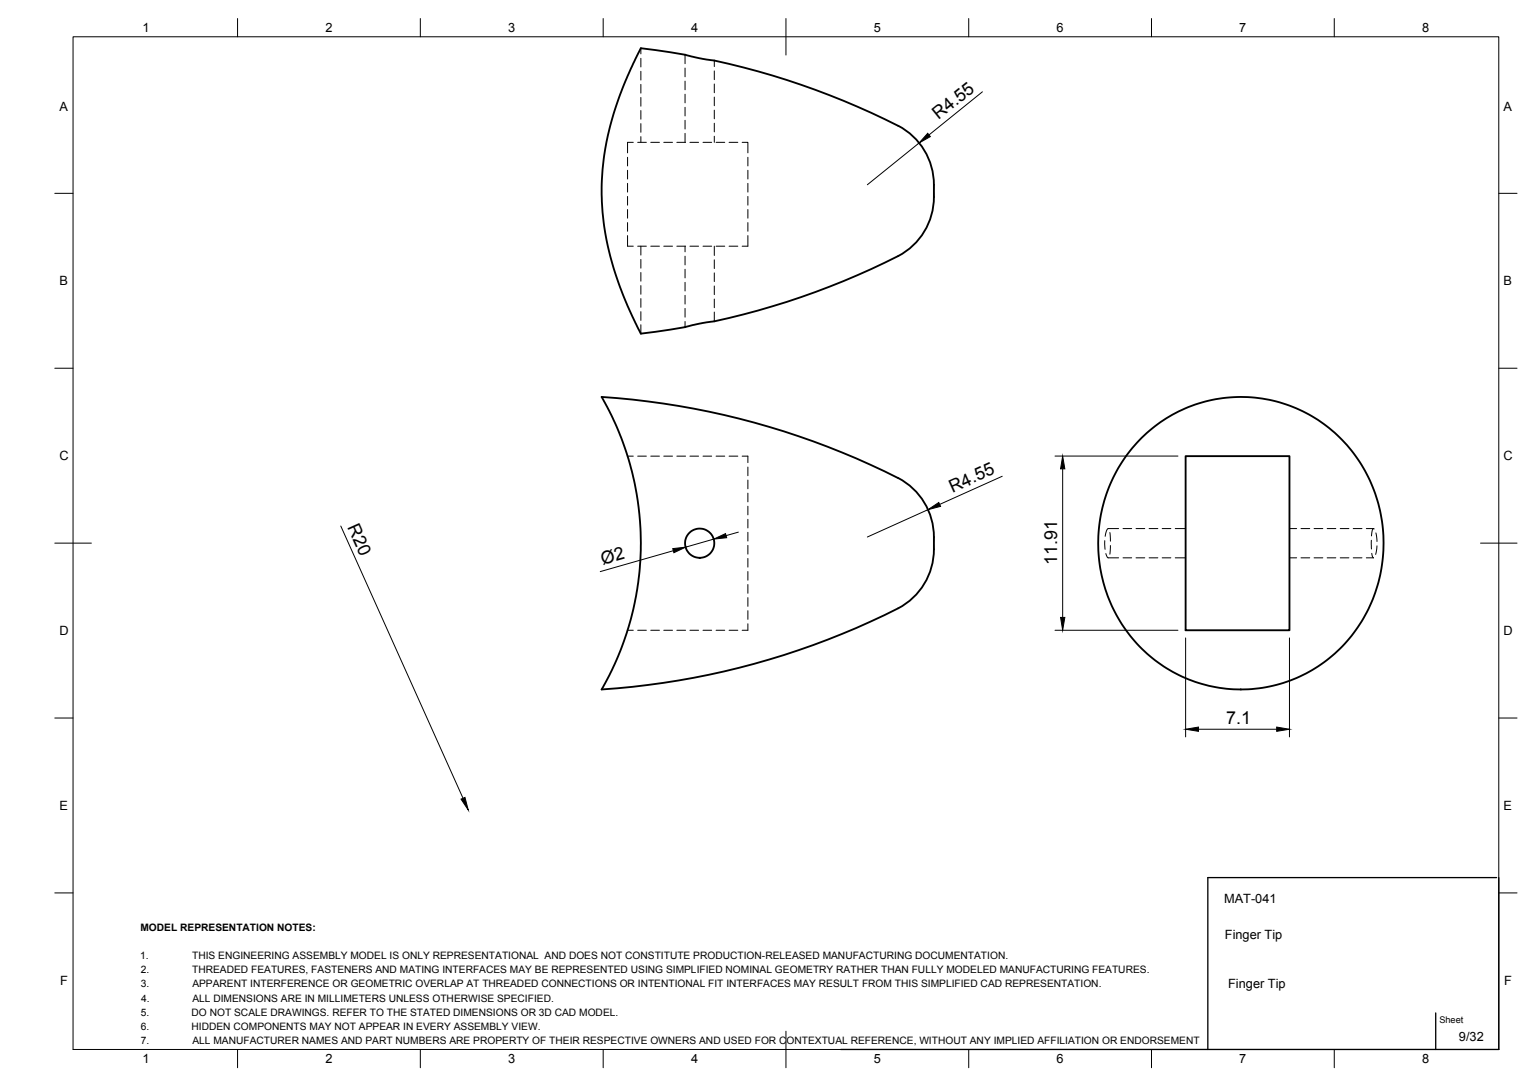
ISO-10303-21;
HEADER;
/* Generated by software containing ST-Developer
 * from STEP Tools, Inc. (www.steptools.com) 
 */

FILE_DESCRIPTION(
/* description */ ('STEP AP214'),
/* implementation_level */ '2;1');

FILE_NAME(
/* name */ 'Finger Tip.step',
/* time_stamp */ '2026-11-14T21:57:47-08:00',
/* author */ (''),
/* organization */ (''),
/* preprocessor_version */ 'ST-DEVELOPER v20.2',
/* originating_system */ 'Autodesk Translation Framework v15.17.0.0',
/* authorisation */ '');

FILE_SCHEMA (('AUTOMOTIVE_DESIGN { 1 0 10303 214 3 1 1 }'));
ENDSEC;

DATA;
#10=MECHANICAL_DESIGN_GEOMETRIC_PRESENTATION_REPRESENTATION('',(#259),#13199);
#11=(
BOUNDED_CURVE()
B_SPLINE_CURVE(2,(#12139,#12140,#12141),.UNSPECIFIED.,.F.,.F.)
B_SPLINE_CURVE_WITH_KNOTS((3,3),(0.0658194535624849,0.468554524158603),
 .UNSPECIFIED.)
CURVE()
GEOMETRIC_REPRESENTATION_ITEM()
RATIONAL_B_SPLINE_CURVE((0.999935484054137,0.979761934520674,1.))
REPRESENTATION_ITEM('')
);
#17=(
BOUNDED_SURFACE()
B_SPLINE_SURFACE(2,2,((#12039,#12040,#12041,#12042,#12043,#12044,#12045,
#12046,#12047),(#12048,#12049,#12050,#12051,#12052,#12053,#12054,#12055,
#12056),(#12057,#12058,#12059,#12060,#12061,#12062,#12063,#12064,#12065)),
 .UNSPECIFIED.,.F.,.T.,.F.)
B_SPLINE_SURFACE_WITH_KNOTS((3,3),(3,2,2,2,3),(-1.66348996389916,-0.482485072527983),
(-3.14159265358979,-1.5707963267949,0.,1.5707963267949,3.14159265358979),
 .UNSPECIFIED.)
GEOMETRIC_REPRESENTATION_ITEM()
RATIONAL_B_SPLINE_SURFACE(((1.,0.707106781186548,1.,0.707106781186548,1.,
0.707106781186548,1.,0.707106781186548,1.),(0.830661033030149,0.587366049323041,
0.830661033030149,0.587366049323041,0.830661033030149,0.587366049323041,
0.830661033030149,0.587366049323041,0.830661033030149),(1.,0.707106781186548,
1.,0.707106781186548,1.,0.707106781186548,1.,0.707106781186548,1.)))
REPRESENTATION_ITEM('')
SURFACE()
);
#18=(
BOUNDED_SURFACE()
B_SPLINE_SURFACE(2,2,((#12070,#12071,#12072,#12073,#12074,#12075,#12076,
#12077,#12078),(#12079,#12080,#12081,#12082,#12083,#12084,#12085,#12086,
#12087),(#12088,#12089,#12090,#12091,#12092,#12093,#12094,#12095,#12096)),
 .UNSPECIFIED.,.F.,.T.,.F.)
B_SPLINE_SURFACE_WITH_KNOTS((3,3),(3,2,2,2,3),(-0.468554524158603,-0.0651764989564067),
(-3.14159265358979,-1.5707963267949,0.,1.5707963267949,3.14159265358979),
 .UNSPECIFIED.)
GEOMETRIC_REPRESENTATION_ITEM()
RATIONAL_B_SPLINE_SURFACE(((1.,0.707106781186548,1.,0.707106781186548,1.,
0.707106781186548,1.,0.707106781186548,1.),(0.979729625048845,0.692773461601392,
0.979729625048845,0.692773461601392,0.979729625048845,0.692773461601392,
0.979729625048845,0.692773461601392,0.979729625048845),(1.,0.707106781186548,
1.,0.707106781186548,1.,0.707106781186548,1.,0.707106781186548,1.)))
REPRESENTATION_ITEM('')
SURFACE()
);
#184=B_SPLINE_CURVE_WITH_KNOTS('',3,(#11947,#11948,#11949,#11950,#11951,
#11952,#11953,#11954,#11955,#11956,#11957,#11958,#11959,#11960,#11961,#11962,
#11963,#11964,#11965,#11966,#11967,#11968,#11969),.UNSPECIFIED.,.F.,.F.,
(4,2,2,2,2,3,2,2,2,2,4),(0.476645491037206,0.489023957516382,0.527166589495669,
0.568095012367448,0.607142264956957,0.636252225893218,0.674200453389387,
0.713373161852222,0.750226922703377,0.78797801482852,0.795881712617993),
 .UNSPECIFIED.);
#185=B_SPLINE_CURVE_WITH_KNOTS('',3,(#11970,#11971,#11972,#11973,#11974,
#11975,#11976,#11977,#11978,#11979,#11980,#11981,#11982,#11983,#11984,#11985,
#11986,#11987,#11988,#11989),.UNSPECIFIED.,.F.,.F.,(4,2,2,2,2,2,2,2,2,4),
(0.159629486724776,0.18739470215505,0.223766252646954,0.263805807870951,
0.302029537123351,0.34097527431584,0.380812071035441,0.417115871073174,
0.453232846571769,0.476645491037206),.UNSPECIFIED.);
#186=B_SPLINE_CURVE_WITH_KNOTS('',3,(#11993,#11994,#11995,#11996,#11997,
#11998,#11999,#12000,#12001,#12002,#12003,#12004,#12005,#12006,#12007,#12008,
#12009,#12010,#12011,#12012,#12013,#12014,#12015),.UNSPECIFIED.,.F.,.F.,
(4,2,2,2,2,3,2,2,2,2,4),(0.476645491037025,0.48902395751638,0.527166589495666,
0.568095012367448,0.607142264956952,0.636252225893214,0.674200453389384,
0.713373161852219,0.75022692270337,0.78797801482851,0.795881712618303),
 .UNSPECIFIED.);
#187=B_SPLINE_CURVE_WITH_KNOTS('',3,(#12019,#12020,#12021,#12022,#12023,
#12024,#12025,#12026,#12027,#12028,#12029,#12030,#12031,#12032,#12033,#12034,
#12035,#12036,#12037,#12038),.UNSPECIFIED.,.F.,.F.,(4,2,2,2,2,2,2,2,2,4),
(0.795881712618303,0.823646928048259,0.860018478540157,0.900058033764149,
0.938281763016554,0.977227500209047,1.01706429692865,1.05336809696638,1.08948507246498,
1.11289771693024),.UNSPECIFIED.);
#188=B_SPLINE_CURVE_WITH_KNOTS('',3,(#12098,#12099,#12100,#12101,#12102,
#12103,#12104,#12105,#12106,#12107,#12108,#12109,#12110,#12111,#12112,#12113,
#12114,#12115,#12116,#12117,#12118,#12119,#12120,#12121,#12122,#12123,#12124,
#12125,#12126,#12127,#12128,#12129,#12130,#12131,#12132,#12133,#12134,#12135,
#12136,#12137,#12138),.UNSPECIFIED.,.T.,.F.,(4,2,2,2,2,2,3,2,2,2,2,2,2,
2,2,2,2,2,2,4),(4.76570010814283,4.82373748195937,5.15211023194195,5.51811468114358,
5.92483477190322,6.13853392596326,6.35204429850806,6.71291359634487,7.09425816350559,
7.50552237110612,7.8592853831874,8.18933065337909,8.53450621361463,8.93047115205954,
9.32063251608662,9.68763081499438,10.0531628494056,10.4503791856812,10.8359489090294,
11.1177444066509),.UNSPECIFIED.);
#223=SHAPE_REPRESENTATION_RELATIONSHIP('SRR','None',#13294,#241);
#241=ADVANCED_BREP_SHAPE_REPRESENTATION('',(#277),#13190);
#259=STYLED_ITEM('',(#13409),#277);
#277=MANIFOLD_SOLID_BREP('Body1',#6854);
#349=FACE_BOUND('',#2535,.T.);
#350=FACE_BOUND('',#2536,.T.);
#351=FACE_BOUND('',#2538,.T.);
#352=FACE_BOUND('',#2542,.T.);
#353=FACE_BOUND('',#2545,.T.);
#538=PLANE('',#7605);
#539=PLANE('',#7606);
#540=PLANE('',#7607);
#541=PLANE('',#7608);
#542=PLANE('',#7609);
#968=LINE('',#11945,#1486);
#969=LINE('',#12017,#1487);
#970=LINE('',#12147,#1488);
#971=LINE('',#12150,#1489);
#972=LINE('',#12154,#1490);
#973=LINE('',#12156,#1491);
#974=LINE('',#12158,#1492);
#975=LINE('',#12159,#1493);
#976=LINE('',#12161,#1494);
#977=LINE('',#12162,#1495);
#978=LINE('',#12164,#1496);
#979=LINE('',#12166,#1497);
#1486=VECTOR('',#9263,1.);
#1487=VECTOR('',#9266,1.);
#1488=VECTOR('',#9277,1000.);
#1489=VECTOR('',#9280,1000.);
#1490=VECTOR('',#9283,1000.);
#1491=VECTOR('',#9284,1000.);
#1492=VECTOR('',#9285,1000.);
#1493=VECTOR('',#9286,1000.);
#1494=VECTOR('',#9289,1000.);
#1495=VECTOR('',#9290,1000.);
#1496=VECTOR('',#9293,1000.);
#1497=VECTOR('',#9296,1000.);
#1754=CYLINDRICAL_SURFACE('',#7596,1.);
#1755=CYLINDRICAL_SURFACE('',#7598,1.);
#1756=CYLINDRICAL_SURFACE('',#7602,20.);
#2075=FACE_OUTER_BOUND('',#2531,.T.);
#2076=FACE_OUTER_BOUND('',#2532,.T.);
#2077=FACE_OUTER_BOUND('',#2533,.T.);
#2078=FACE_OUTER_BOUND('',#2534,.T.);
#2079=FACE_OUTER_BOUND('',#2537,.T.);
#2080=FACE_OUTER_BOUND('',#2539,.T.);
#2081=FACE_OUTER_BOUND('',#2540,.T.);
#2082=FACE_OUTER_BOUND('',#2541,.T.);
#2083=FACE_OUTER_BOUND('',#2543,.T.);
#2084=FACE_OUTER_BOUND('',#2544,.T.);
#2531=EDGE_LOOP('',(#5862,#5863,#5864,#5865,#5866));
#2532=EDGE_LOOP('',(#5867,#5868,#5869,#5870,#5871));
#2533=EDGE_LOOP('',(#5872,#5873,#5874));
#2534=EDGE_LOOP('',(#5875,#5876,#5877,#5878));
#2535=EDGE_LOOP('',(#5879,#5880));
#2536=EDGE_LOOP('',(#5881,#5882));
#2537=EDGE_LOOP('',(#5883));
#2538=EDGE_LOOP('',(#5884,#5885,#5886,#5887));
#2539=EDGE_LOOP('',(#5888,#5889,#5890,#5891));
#2540=EDGE_LOOP('',(#5892,#5893,#5894,#5895));
#2541=EDGE_LOOP('',(#5896,#5897,#5898,#5899));
#2542=EDGE_LOOP('',(#5900));
#2543=EDGE_LOOP('',(#5901,#5902,#5903,#5904));
#2544=EDGE_LOOP('',(#5905,#5906,#5907,#5908));
#2545=EDGE_LOOP('',(#5909));
#2909=CIRCLE('',#7597,1.);
#2910=CIRCLE('',#7599,1.);
#2911=CIRCLE('',#7600,4.44993914281691);
#2912=CIRCLE('',#7601,4.54815386259491);
#2913=CIRCLE('',#7603,20.);
#2914=CIRCLE('',#7604,20.);
#3422=VERTEX_POINT('',#11942);
#3423=VERTEX_POINT('',#11944);
#3424=VERTEX_POINT('',#11946);
#3425=VERTEX_POINT('',#11991);
#3426=VERTEX_POINT('',#11992);
#3427=VERTEX_POINT('',#12016);
#3428=VERTEX_POINT('',#12066);
#3429=VERTEX_POINT('',#12068);
#3430=VERTEX_POINT('',#12097);
#3431=VERTEX_POINT('',#12143);
#3432=VERTEX_POINT('',#12144);
#3433=VERTEX_POINT('',#12146);
#3434=VERTEX_POINT('',#12148);
#3435=VERTEX_POINT('',#12152);
#3436=VERTEX_POINT('',#12153);
#3437=VERTEX_POINT('',#12155);
#3438=VERTEX_POINT('',#12157);
#4268=EDGE_CURVE('',#3422,#3422,#2909,.T.);
#4269=EDGE_CURVE('',#3422,#3423,#968,.T.);
#4270=EDGE_CURVE('',#3423,#3424,#184,.T.);
#4271=EDGE_CURVE('',#3424,#3423,#185,.T.);
#4272=EDGE_CURVE('',#3425,#3426,#186,.T.);
#4273=EDGE_CURVE('',#3426,#3427,#969,.T.);
#4274=EDGE_CURVE('',#3427,#3427,#2910,.T.);
#4275=EDGE_CURVE('',#3426,#3425,#187,.T.);
#4276=EDGE_CURVE('',#3428,#3428,#2911,.T.);
#4277=EDGE_CURVE('',#3428,#3429,#2912,.T.);
#4278=EDGE_CURVE('',#3430,#3430,#188,.T.);
#4279=EDGE_CURVE('',#3430,#3428,#11,.T.);
#4280=EDGE_CURVE('',#3431,#3432,#2913,.T.);
#4281=EDGE_CURVE('',#3432,#3433,#970,.T.);
#4282=EDGE_CURVE('',#3433,#3434,#2914,.T.);
#4283=EDGE_CURVE('',#3434,#3431,#971,.T.);
#4284=EDGE_CURVE('',#3435,#3436,#972,.T.);
#4285=EDGE_CURVE('',#3436,#3437,#973,.T.);
#4286=EDGE_CURVE('',#3437,#3438,#974,.T.);
#4287=EDGE_CURVE('',#3438,#3435,#975,.T.);
#4288=EDGE_CURVE('',#3437,#3434,#976,.T.);
#4289=EDGE_CURVE('',#3436,#3431,#977,.T.);
#4290=EDGE_CURVE('',#3438,#3433,#978,.T.);
#4291=EDGE_CURVE('',#3435,#3432,#979,.T.);
#5862=ORIENTED_EDGE('',*,*,#4268,.T.);
#5863=ORIENTED_EDGE('',*,*,#4269,.T.);
#5864=ORIENTED_EDGE('',*,*,#4270,.T.);
#5865=ORIENTED_EDGE('',*,*,#4271,.T.);
#5866=ORIENTED_EDGE('',*,*,#4269,.F.);
#5867=ORIENTED_EDGE('',*,*,#4272,.T.);
#5868=ORIENTED_EDGE('',*,*,#4273,.T.);
#5869=ORIENTED_EDGE('',*,*,#4274,.T.);
#5870=ORIENTED_EDGE('',*,*,#4273,.F.);
#5871=ORIENTED_EDGE('',*,*,#4275,.T.);
#5872=ORIENTED_EDGE('',*,*,#4276,.F.);
#5873=ORIENTED_EDGE('',*,*,#4277,.T.);
#5874=ORIENTED_EDGE('',*,*,#4277,.F.);
#5875=ORIENTED_EDGE('',*,*,#4278,.F.);
#5876=ORIENTED_EDGE('',*,*,#4279,.T.);
#5877=ORIENTED_EDGE('',*,*,#4276,.T.);
#5878=ORIENTED_EDGE('',*,*,#4279,.F.);
#5879=ORIENTED_EDGE('',*,*,#4271,.F.);
#5880=ORIENTED_EDGE('',*,*,#4270,.F.);
#5881=ORIENTED_EDGE('',*,*,#4272,.F.);
#5882=ORIENTED_EDGE('',*,*,#4275,.F.);
#5883=ORIENTED_EDGE('',*,*,#4278,.T.);
#5884=ORIENTED_EDGE('',*,*,#4280,.T.);
#5885=ORIENTED_EDGE('',*,*,#4281,.T.);
#5886=ORIENTED_EDGE('',*,*,#4282,.T.);
#5887=ORIENTED_EDGE('',*,*,#4283,.T.);
#5888=ORIENTED_EDGE('',*,*,#4284,.T.);
#5889=ORIENTED_EDGE('',*,*,#4285,.T.);
#5890=ORIENTED_EDGE('',*,*,#4286,.T.);
#5891=ORIENTED_EDGE('',*,*,#4287,.T.);
#5892=ORIENTED_EDGE('',*,*,#4283,.F.);
#5893=ORIENTED_EDGE('',*,*,#4288,.F.);
#5894=ORIENTED_EDGE('',*,*,#4285,.F.);
#5895=ORIENTED_EDGE('',*,*,#4289,.T.);
#5896=ORIENTED_EDGE('',*,*,#4282,.F.);
#5897=ORIENTED_EDGE('',*,*,#4290,.F.);
#5898=ORIENTED_EDGE('',*,*,#4286,.F.);
#5899=ORIENTED_EDGE('',*,*,#4288,.T.);
#5900=ORIENTED_EDGE('',*,*,#4268,.F.);
#5901=ORIENTED_EDGE('',*,*,#4281,.F.);
#5902=ORIENTED_EDGE('',*,*,#4291,.F.);
#5903=ORIENTED_EDGE('',*,*,#4287,.F.);
#5904=ORIENTED_EDGE('',*,*,#4290,.T.);
#5905=ORIENTED_EDGE('',*,*,#4280,.F.);
#5906=ORIENTED_EDGE('',*,*,#4289,.F.);
#5907=ORIENTED_EDGE('',*,*,#4284,.F.);
#5908=ORIENTED_EDGE('',*,*,#4291,.T.);
#5909=ORIENTED_EDGE('',*,*,#4274,.F.);
#6727=ADVANCED_FACE('',(#2075),#1754,.F.);
#6728=ADVANCED_FACE('',(#2076),#1755,.F.);
#6729=ADVANCED_FACE('',(#2077),#17,.F.);
#6730=ADVANCED_FACE('',(#2078,#349,#350),#18,.F.);
#6731=ADVANCED_FACE('',(#2079,#351),#1756,.F.);
#6732=ADVANCED_FACE('',(#2080),#538,.T.);
#6733=ADVANCED_FACE('',(#2081),#539,.F.);
#6734=ADVANCED_FACE('',(#2082,#352),#540,.F.);
#6735=ADVANCED_FACE('',(#2083),#541,.F.);
#6736=ADVANCED_FACE('',(#2084,#353),#542,.F.);
#6854=CLOSED_SHELL('',(#6727,#6728,#6729,#6730,#6731,#6732,#6733,#6734,
#6735,#6736));
#7595=AXIS2_PLACEMENT_3D('',#11940,#9257,#9258);
#7596=AXIS2_PLACEMENT_3D('',#11941,#9259,#9260);
#7597=AXIS2_PLACEMENT_3D('',#11943,#9261,#9262);
#7598=AXIS2_PLACEMENT_3D('',#11990,#9264,#9265);
#7599=AXIS2_PLACEMENT_3D('',#12018,#9267,#9268);
#7600=AXIS2_PLACEMENT_3D('',#12067,#9269,#9270);
#7601=AXIS2_PLACEMENT_3D('',#12069,#9271,#9272);
#7602=AXIS2_PLACEMENT_3D('',#12142,#9273,#9274);
#7603=AXIS2_PLACEMENT_3D('',#12145,#9275,#9276);
#7604=AXIS2_PLACEMENT_3D('',#12149,#9278,#9279);
#7605=AXIS2_PLACEMENT_3D('',#12151,#9281,#9282);
#7606=AXIS2_PLACEMENT_3D('',#12160,#9287,#9288);
#7607=AXIS2_PLACEMENT_3D('',#12163,#9291,#9292);
#7608=AXIS2_PLACEMENT_3D('',#12165,#9294,#9295);
#7609=AXIS2_PLACEMENT_3D('',#12167,#9297,#9298);
#9257=DIRECTION('axis',(0.,0.,1.));
#9258=DIRECTION('refdir',(1.,0.,0.));
#9259=DIRECTION('center_axis',(-1.,0.,0.));
#9260=DIRECTION('ref_axis',(0.,0.,1.));
#9261=DIRECTION('center_axis',(1.,0.,3.64131712001849E-16));
#9262=DIRECTION('ref_axis',(-3.64131712001849E-16,0.,1.));
#9263=DIRECTION('',(-1.,0.,0.));
#9264=DIRECTION('center_axis',(-1.,0.,0.));
#9265=DIRECTION('ref_axis',(0.,0.,1.));
#9266=DIRECTION('',(-1.,0.,0.));
#9267=DIRECTION('center_axis',(-1.,0.,-2.91305369601479E-16));
#9268=DIRECTION('ref_axis',(2.91305369601479E-16,0.,-1.));
#9269=DIRECTION('center_axis',(0.,-1.,0.));
#9270=DIRECTION('ref_axis',(0.,0.,-1.));
#9271=DIRECTION('center_axis',(-1.,0.,-2.23423785287372E-16));
#9272=DIRECTION('ref_axis',(-2.23423785287372E-16,0.,1.));
#9273=DIRECTION('center_axis',(-1.,0.,0.));
#9274=DIRECTION('ref_axis',(0.,0.,1.));
#9275=DIRECTION('center_axis',(-1.,0.,-2.91305369601479E-16));
#9276=DIRECTION('ref_axis',(2.91305369601479E-16,-1.73472347597681E-15,
-1.));
#9277=DIRECTION('',(-1.,0.,0.));
#9278=DIRECTION('center_axis',(1.,0.,3.64131712001849E-16));
#9279=DIRECTION('ref_axis',(-3.64131712001849E-16,-3.46944695195361E-15,
1.));
#9280=DIRECTION('',(1.,0.,0.));
#9281=DIRECTION('center_axis',(0.,-1.,0.));
#9282=DIRECTION('ref_axis',(0.,0.,-1.));
#9283=DIRECTION('',(-2.91305369601479E-16,0.,1.));
#9284=DIRECTION('',(-1.,0.,0.));
#9285=DIRECTION('',(3.64131712001849E-16,0.,-1.));
#9286=DIRECTION('',(1.,0.,0.));
#9287=DIRECTION('center_axis',(0.,0.,1.));
#9288=DIRECTION('ref_axis',(1.,0.,0.));
#9289=DIRECTION('',(0.,-1.,0.));
#9290=DIRECTION('',(0.,-1.,0.));
#9291=DIRECTION('center_axis',(-1.,0.,-3.64131712001849E-16));
#9292=DIRECTION('ref_axis',(-3.64131712001849E-16,0.,1.));
#9293=DIRECTION('',(0.,-1.,0.));
#9294=DIRECTION('center_axis',(0.,0.,-1.));
#9295=DIRECTION('ref_axis',(-1.,0.,0.));
#9296=DIRECTION('',(0.,-1.,0.));
#9297=DIRECTION('center_axis',(1.,0.,2.91305369601479E-16));
#9298=DIRECTION('ref_axis',(2.91305369601479E-16,0.,-1.));
#11940=CARTESIAN_POINT('',(0.,0.,0.));
#11941=CARTESIAN_POINT('Origin',(26.,6.7016908093449,-4.06575814682064E-16));
#11942=CARTESIAN_POINT('',(6.67681390339618,6.7016908093449,-1.));
#11943=CARTESIAN_POINT('Origin',(6.67681390339618,6.7016908093449,-4.06575814682064E-16));
#11944=CARTESIAN_POINT('',(0.932251906823188,6.7016908093449,-1.));
#11945=CARTESIAN_POINT('',(26.,6.7016908093449,-1.));
#11946=CARTESIAN_POINT('',(0.932251906822564,6.70169080934177,1.));
#11947=CARTESIAN_POINT('Ctrl Pts',(0.932251906823183,6.70169080934491,-1.));
#11948=CARTESIAN_POINT('Ctrl Pts',(0.924248549049917,6.66131091017121,-1.));
#11949=CARTESIAN_POINT('Ctrl Pts',(0.916026356968957,6.62094102048031,-0.997554276745439));
#11950=CARTESIAN_POINT('Ctrl Pts',(0.881783128220109,6.45711744573232,-0.977603465009505));
#11951=CARTESIAN_POINT('Ctrl Pts',(0.854654659643743,6.33738348753352,-0.939561735078518));
#11952=CARTESIAN_POINT('Ctrl Pts',(0.800113400469254,6.11014608328131,-0.817261967795165));
#11953=CARTESIAN_POINT('Ctrl Pts',(0.77328444103289,6.00592553072582,-0.730775745996131));
#11954=CARTESIAN_POINT('Ctrl Pts',(0.729480326144063,5.8413149278795,-0.525593218279249));
#11955=CARTESIAN_POINT('Ctrl Pts',(0.712545126681715,5.78058813656252,-0.410370125980672));
#11956=CARTESIAN_POINT('Ctrl Pts',(0.694345193897906,5.71580700056676,-0.193362294484071));
#11957=CARTESIAN_POINT('Ctrl Pts',(0.690307391982312,5.70169080934487,-0.0970332031208705));
#11958=CARTESIAN_POINT('Ctrl Pts',(0.690307391982312,5.70169080934487,-5.70054262672731E-16));
#11959=CARTESIAN_POINT('Ctrl Pts',(0.690307391982312,5.70169080934487,0.126494091653897));
#11960=CARTESIAN_POINT('Ctrl Pts',(0.697192186740198,5.72567100919992,0.25144246077573));
#11961=CARTESIAN_POINT('Ctrl Pts',(0.723443573443553,5.81990229608856,0.48920911768999));
#11962=CARTESIAN_POINT('Ctrl Pts',(0.742874919145282,5.89055183127276,0.598815192100498));
#11963=CARTESIAN_POINT('Ctrl Pts',(0.787956450068906,6.06311917062026,0.779008106316694));
#11964=CARTESIAN_POINT('Ctrl Pts',(0.812798404624451,6.16166185353399,0.85019109475144));
#11965=CARTESIAN_POINT('Ctrl Pts',(0.864691942139612,6.38122379163014,0.955232747406083));
#11966=CARTESIAN_POINT('Ctrl Pts',(0.891412884359187,6.50130511642615,0.987456747739729));
#11967=CARTESIAN_POINT('Ctrl Pts',(0.921933001916271,6.65008201775339,0.999001452378396));
#11968=CARTESIAN_POINT('Ctrl Pts',(0.927138034517321,6.67588943272924,0.999999999999919));
#11969=CARTESIAN_POINT('Ctrl Pts',(0.93225190682257,6.70169080934177,1.));
#11970=CARTESIAN_POINT('Ctrl Pts',(0.93225190682257,6.70169080934177,1.));
#11971=CARTESIAN_POINT('Ctrl Pts',(0.95021663295712,6.7923294950717,1.00000000000028));
#11972=CARTESIAN_POINT('Ctrl Pts',(0.967037947810111,6.88289731649557,0.987678651235166));
#11973=CARTESIAN_POINT('Ctrl Pts',(1.00234665201365,7.08612514530952,0.930876070129687));
#11974=CARTESIAN_POINT('Ctrl Pts',(1.01939410567033,7.19503949676066,0.87813724044672));
#11975=CARTESIAN_POINT('Ctrl Pts',(1.04879439681428,7.39931145844304,0.728642051211854));
#11976=CARTESIAN_POINT('Ctrl Pts',(1.06022559732792,7.48994901935284,0.629606965290707));
#11977=CARTESIAN_POINT('Ctrl Pts',(1.07617030128948,7.62419484684745,0.406408985865648));
#11978=CARTESIAN_POINT('Ctrl Pts',(1.08086902511051,7.66842539636241,0.285763077415728));
#11979=CARTESIAN_POINT('Ctrl Pts',(1.0852457498272,7.70958096263185,0.0318261665609532));
#11980=CARTESIAN_POINT('Ctrl Pts',(1.08480714142453,7.70519119859556,-0.0991848216234942));
#11981=CARTESIAN_POINT('Ctrl Pts',(1.07843262498588,7.645938513344,-0.355002569322465));
#11982=CARTESIAN_POINT('Ctrl Pts',(1.07240914531565,7.59053680524487,-0.476976092322022));
#11983=CARTESIAN_POINT('Ctrl Pts',(1.05418970048312,7.44253010180747,-0.682447869986455));
#11984=CARTESIAN_POINT('Ctrl Pts',(1.04269942111853,7.35498368680039,-0.766583478682305));
#11985=CARTESIAN_POINT('Ctrl Pts',(1.0132565948215,7.15527406689819,-0.899197300474265));
#11986=CARTESIAN_POINT('Ctrl Pts',(0.995565232471033,7.0450187623199,-0.946689410696543));
#11987=CARTESIAN_POINT('Ctrl Pts',(0.961736774919552,6.85447725024748,-0.991251376980505));
#11988=CARTESIAN_POINT('Ctrl Pts',(0.947389466099236,6.7780653929409,-1.));
#11989=CARTESIAN_POINT('Ctrl Pts',(0.932251906823183,6.70169080934491,-1.));
#11990=CARTESIAN_POINT('Origin',(26.,6.7016908093449,-4.06575814682064E-16));
#11991=CARTESIAN_POINT('',(19.0677480931767,6.70169080934559,1.));
#11992=CARTESIAN_POINT('',(19.0677480931768,6.7016908093449,-1.));
#11993=CARTESIAN_POINT('Ctrl Pts',(19.0677480931765,6.70169080934669,1.));
#11994=CARTESIAN_POINT('Ctrl Pts',(19.0757514509498,6.6613109101724,1.00000000000007));
#11995=CARTESIAN_POINT('Ctrl Pts',(19.0839736430309,6.62094102048092,0.997554276745514));
#11996=CARTESIAN_POINT('Ctrl Pts',(19.1182168717799,6.45711744573232,0.977603465009509));
#11997=CARTESIAN_POINT('Ctrl Pts',(19.1453453403563,6.3373834875335,0.939561735078495));
#11998=CARTESIAN_POINT('Ctrl Pts',(19.1998865995307,6.11014608328137,0.817261967795189));
#11999=CARTESIAN_POINT('Ctrl Pts',(19.2267155589671,6.00592553072585,0.730775745996161));
#12000=CARTESIAN_POINT('Ctrl Pts',(19.2705196738559,5.84131492787951,0.525593218279265));
#12001=CARTESIAN_POINT('Ctrl Pts',(19.2874548733183,5.78058813656252,0.410370125980689));
#12002=CARTESIAN_POINT('Ctrl Pts',(19.3056548061021,5.71580700056676,0.193362294484076));
#12003=CARTESIAN_POINT('Ctrl Pts',(19.3096926080177,5.70169080934487,0.0970332031208726));
#12004=CARTESIAN_POINT('Ctrl Pts',(19.3096926080177,5.70169080934487,-5.70054262672731E-16));
#12005=CARTESIAN_POINT('Ctrl Pts',(19.3096926080177,5.70169080934487,-0.126494091653898));
#12006=CARTESIAN_POINT('Ctrl Pts',(19.3028078132598,5.72567100919992,-0.251442460775731));
#12007=CARTESIAN_POINT('Ctrl Pts',(19.2765564265564,5.81990229608856,-0.489209117689992));
#12008=CARTESIAN_POINT('Ctrl Pts',(19.2571250808547,5.89055183127276,-0.598815192100501));
#12009=CARTESIAN_POINT('Ctrl Pts',(19.2120435499311,6.06311917062025,-0.779008106316688));
#12010=CARTESIAN_POINT('Ctrl Pts',(19.1872015953756,6.16166185353397,-0.850191094751436));
#12011=CARTESIAN_POINT('Ctrl Pts',(19.1353080578604,6.38122379163016,-0.955232747406096));
#12012=CARTESIAN_POINT('Ctrl Pts',(19.1085871156408,6.50130511642616,-0.987456747739731));
#12013=CARTESIAN_POINT('Ctrl Pts',(19.0780669980835,6.65008201775443,-0.999001452378478));
#12014=CARTESIAN_POINT('Ctrl Pts',(19.0728619654823,6.67588943273133,-1.));
#12015=CARTESIAN_POINT('Ctrl Pts',(19.0677480931768,6.7016908093449,-1.));
#12016=CARTESIAN_POINT('',(13.7768139033962,6.7016908093449,-1.));
#12017=CARTESIAN_POINT('',(26.,6.7016908093449,-1.));
#12018=CARTESIAN_POINT('Origin',(13.7768139033962,6.7016908093449,-4.06575814682064E-16));
#12019=CARTESIAN_POINT('Ctrl Pts',(19.0677480931768,6.7016908093449,-1.));
#12020=CARTESIAN_POINT('Ctrl Pts',(19.0497833670425,6.79232949507379,-1.));
#12021=CARTESIAN_POINT('Ctrl Pts',(19.0329620521897,6.88289731649658,-0.987678651234883));
#12022=CARTESIAN_POINT('Ctrl Pts',(18.9976533479864,7.08612514530949,-0.930876070129694));
#12023=CARTESIAN_POINT('Ctrl Pts',(18.9806058943297,7.19503949676065,-0.878137240446731));
#12024=CARTESIAN_POINT('Ctrl Pts',(18.9512056031857,7.39931145844305,-0.728642051211849));
#12025=CARTESIAN_POINT('Ctrl Pts',(18.9397744026721,7.48994901935284,-0.629606965290706));
#12026=CARTESIAN_POINT('Ctrl Pts',(18.9238296987105,7.62419484684746,-0.40640898586564));
#12027=CARTESIAN_POINT('Ctrl Pts',(18.9191309748895,7.66842539636241,-0.285763077415725));
#12028=CARTESIAN_POINT('Ctrl Pts',(18.9147542501728,7.70958096263184,-0.0318261665609708));
#12029=CARTESIAN_POINT('Ctrl Pts',(18.9151928585755,7.70519119859557,0.0991848216234665));
#12030=CARTESIAN_POINT('Ctrl Pts',(18.9215673750141,7.64593851334401,0.355002569322444));
#12031=CARTESIAN_POINT('Ctrl Pts',(18.9275908546843,7.59053680524489,0.476976092321998));
#12032=CARTESIAN_POINT('Ctrl Pts',(18.9458102995169,7.44253010180748,0.682447869986442));
#12033=CARTESIAN_POINT('Ctrl Pts',(18.9573005788815,7.3549836868004,0.766583478682293));
#12034=CARTESIAN_POINT('Ctrl Pts',(18.9867434051785,7.1552740668982,0.89919730047426));
#12035=CARTESIAN_POINT('Ctrl Pts',(19.004434767529,7.0450187623199,0.946689410696536));
#12036=CARTESIAN_POINT('Ctrl Pts',(19.0382632250803,6.85447725024808,0.991251376980361));
#12037=CARTESIAN_POINT('Ctrl Pts',(19.0526105339005,6.77806539294211,0.999999999999863));
#12038=CARTESIAN_POINT('Ctrl Pts',(19.0677480931765,6.70169080934669,1.));
#12039=CARTESIAN_POINT('Ctrl Pts',(10.,22.6942090407623,-1.38777878078145E-16));
#12040=CARTESIAN_POINT('Ctrl Pts',(10.,22.6942090407623,-1.38777878078145E-16));
#12041=CARTESIAN_POINT('Ctrl Pts',(10.,22.6942090407623,0.));
#12042=CARTESIAN_POINT('Ctrl Pts',(10.,22.6942090407623,1.38777878078145E-16));
#12043=CARTESIAN_POINT('Ctrl Pts',(10.,22.6942090407623,1.38777878078145E-16));
#12044=CARTESIAN_POINT('Ctrl Pts',(10.,22.6942090407623,1.38777878078145E-16));
#12045=CARTESIAN_POINT('Ctrl Pts',(10.,22.6942090407623,0.));
#12046=CARTESIAN_POINT('Ctrl Pts',(10.,22.6942090407623,-1.38777878078145E-16));
#12047=CARTESIAN_POINT('Ctrl Pts',(10.,22.6942090407623,-1.38777878078145E-16));
#12048=CARTESIAN_POINT('Ctrl Pts',(10.,22.9763860067717,3.03546549996621));
#12049=CARTESIAN_POINT('Ctrl Pts',(6.96453450003379,22.9763860067717,3.03546549996621));
#12050=CARTESIAN_POINT('Ctrl Pts',(6.96453450003379,22.9763860067717,0.));
#12051=CARTESIAN_POINT('Ctrl Pts',(6.96453450003379,22.9763860067717,-3.03546549996621));
#12052=CARTESIAN_POINT('Ctrl Pts',(10.,22.9763860067717,-3.03546549996621));
#12053=CARTESIAN_POINT('Ctrl Pts',(13.0354654999662,22.9763860067717,-3.03546549996621));
#12054=CARTESIAN_POINT('Ctrl Pts',(13.0354654999662,22.9763860067717,0.));
#12055=CARTESIAN_POINT('Ctrl Pts',(13.0354654999662,22.9763860067717,3.03546549996621));
#12056=CARTESIAN_POINT('Ctrl Pts',(10.,22.9763860067717,3.03546549996621));
#12057=CARTESIAN_POINT('Ctrl Pts',(10.,20.2758418106305,4.44993914281691));
#12058=CARTESIAN_POINT('Ctrl Pts',(5.55006085718309,20.2758418106305,4.44993914281691));
#12059=CARTESIAN_POINT('Ctrl Pts',(5.55006085718309,20.2758418106305,0.));
#12060=CARTESIAN_POINT('Ctrl Pts',(5.55006085718309,20.2758418106305,-4.44993914281691));
#12061=CARTESIAN_POINT('Ctrl Pts',(10.,20.2758418106305,-4.44993914281691));
#12062=CARTESIAN_POINT('Ctrl Pts',(14.4499391428169,20.2758418106305,-4.44993914281691));
#12063=CARTESIAN_POINT('Ctrl Pts',(14.4499391428169,20.2758418106305,0.));
#12064=CARTESIAN_POINT('Ctrl Pts',(14.4499391428169,20.2758418106305,4.44993914281691));
#12065=CARTESIAN_POINT('Ctrl Pts',(10.,20.2758418106305,4.44993914281691));
#12066=CARTESIAN_POINT('',(10.,20.2758418106305,4.44993914281691));
#12067=CARTESIAN_POINT('Origin',(10.,20.2758418106305,0.));
#12068=CARTESIAN_POINT('',(10.,22.6942090407623,0.));
#12069=CARTESIAN_POINT('Origin',(10.,18.165580311944,0.420981465576021));
#12070=CARTESIAN_POINT('Ctrl Pts',(10.,20.2758418106305,4.44993914281691));
#12071=CARTESIAN_POINT('Ctrl Pts',(5.5500608571831,20.2758418106305,4.4499391428169));
#12072=CARTESIAN_POINT('Ctrl Pts',(5.5500608571831,20.2758418106305,0.));
#12073=CARTESIAN_POINT('Ctrl Pts',(5.5500608571831,20.2758418106305,-4.4499391428169));
#12074=CARTESIAN_POINT('Ctrl Pts',(10.,20.2758418106305,-4.44993914281691));
#12075=CARTESIAN_POINT('Ctrl Pts',(14.4499391428169,20.2758418106305,-4.4499391428169));
#12076=CARTESIAN_POINT('Ctrl Pts',(14.4499391428169,20.2758418106305,0.));
#12077=CARTESIAN_POINT('Ctrl Pts',(14.4499391428169,20.2758418106305,4.4499391428169));
#12078=CARTESIAN_POINT('Ctrl Pts',(10.,20.2758418106305,4.44993914281691));
#12079=CARTESIAN_POINT('Ctrl Pts',(10.,10.6889014672656,9.30235729258629));
#12080=CARTESIAN_POINT('Ctrl Pts',(0.697642707413711,10.6889014672656,9.30235729258629));
#12081=CARTESIAN_POINT('Ctrl Pts',(0.697642707413709,10.6889014672656,0.));
#12082=CARTESIAN_POINT('Ctrl Pts',(0.697642707413711,10.6889014672656,-9.30235729258629));
#12083=CARTESIAN_POINT('Ctrl Pts',(10.,10.6889014672656,-9.30235729258629));
#12084=CARTESIAN_POINT('Ctrl Pts',(19.3023572925863,10.6889014672656,-9.30235729258629));
#12085=CARTESIAN_POINT('Ctrl Pts',(19.3023572925863,10.6889014672656,0.));
#12086=CARTESIAN_POINT('Ctrl Pts',(19.3023572925863,10.6889014672656,9.30235729258629));
#12087=CARTESIAN_POINT('Ctrl Pts',(10.,10.6889014672656,9.30235729258629));
#12088=CARTESIAN_POINT('Ctrl Pts',(10.,-0.0333011709430475,10.0021841516323));
#12089=CARTESIAN_POINT('Ctrl Pts',(-0.00218415163227181,-0.0333011709430475,
10.0021841516323));
#12090=CARTESIAN_POINT('Ctrl Pts',(-0.00218415163227403,-0.0333011709430475,
0.));
#12091=CARTESIAN_POINT('Ctrl Pts',(-0.00218415163227181,-0.0333011709430475,
-10.0021841516323));
#12092=CARTESIAN_POINT('Ctrl Pts',(10.,-0.0333011709430475,-10.0021841516323));
#12093=CARTESIAN_POINT('Ctrl Pts',(20.0021841516323,-0.0333011709430475,
-10.0021841516323));
#12094=CARTESIAN_POINT('Ctrl Pts',(20.0021841516323,-0.0333011709430475,
0.));
#12095=CARTESIAN_POINT('Ctrl Pts',(20.0021841516323,-0.0333011709430475,
10.0021841516323));
#12096=CARTESIAN_POINT('Ctrl Pts',(10.,-0.0333011709430475,10.0021841516323));
#12097=CARTESIAN_POINT('',(9.99999987317287,0.000194077067732489,10.0000928969774));
#12098=CARTESIAN_POINT('Ctrl Pts',(9.99999987317287,0.000194077067732486,
10.0000928969774));
#12099=CARTESIAN_POINT('Ctrl Pts',(9.80810904601693,9.1950696030043E-5,
10.0000442778392));
#12100=CARTESIAN_POINT('Ctrl Pts',(9.61573304980258,0.00331798875440397,
9.99425980218522));
#12101=CARTESIAN_POINT('Ctrl Pts',(8.33291717935469,0.0477168426728619,
9.91718091357786));
#12102=CARTESIAN_POINT('Ctrl Pts',(7.27724454850721,0.193447639956633,9.66841352790813));
#12103=CARTESIAN_POINT('Ctrl Pts',(5.18973500313614,0.649166839307786,8.79546486797327));
#12104=CARTESIAN_POINT('Ctrl Pts',(4.19507286136815,0.969114760287138,8.13936989246473));
#12105=CARTESIAN_POINT('Ctrl Pts',(2.40058556231555,1.64336913807273,6.42724037761097));
#12106=CARTESIAN_POINT('Ctrl Pts',(1.63759314204628,1.99433660295155,5.33756391116479));
#12107=CARTESIAN_POINT('Ctrl Pts',(0.823620674034291,2.38573688258387,3.47744015908405));
#12108=CARTESIAN_POINT('Ctrl Pts',(0.608585489527882,2.49400970267041,2.8055797921226));
#12109=CARTESIAN_POINT('Ctrl Pts',(0.3189262235327,2.64124370193303,1.41915458981438));
#12110=CARTESIAN_POINT('Ctrl Pts',(0.245631819034601,2.67949192431123,0.711701241816013));
#12111=CARTESIAN_POINT('Ctrl Pts',(0.2456318190346,2.67949192431123,5.96744875736022E-15));
#12112=CARTESIAN_POINT('Ctrl Pts',(0.245631819034601,2.67949192431123,-1.20289765945603));
#12113=CARTESIAN_POINT('Ctrl Pts',(0.454406269039078,2.56890479083654,-2.3863380426886));
#12114=CARTESIAN_POINT('Ctrl Pts',(1.28433866991227,2.16096119478927,-4.68032816011342));
#12115=CARTESIAN_POINT('Ctrl Pts',(1.91916845937342,1.85829341673215,-5.75624332867574));
#12116=CARTESIAN_POINT('Ctrl Pts',(3.59440265680175,1.17782954694983,-7.67651894426489));
#12117=CARTESIAN_POINT('Ctrl Pts',(4.65794493564582,0.799305541817284,-8.49042605227953));
#12118=CARTESIAN_POINT('Ctrl Pts',(6.89944797346244,0.256191889285011,-9.55859137985788));
#12119=CARTESIAN_POINT('Ctrl Pts',(8.02464547197843,0.0758487766023874,
-9.86811069108096));
#12120=CARTESIAN_POINT('Ctrl Pts',(10.2891271125017,-0.033299425832443,
-10.0580114046642));
#12121=CARTESIAN_POINT('Ctrl Pts',(11.3784610421618,0.0243895637395715,
-9.96258304339045));
#12122=CARTESIAN_POINT('Ctrl Pts',(13.5297527353772,0.335468227226224,-9.40075939411568));
#12123=CARTESIAN_POINT('Ctrl Pts',(14.5547382087638,0.591005341871764,-8.92516032239902));
#12124=CARTESIAN_POINT('Ctrl Pts',(16.516698088114,1.20843453126161,-7.57040193616715));
#12125=CARTESIAN_POINT('Ctrl Pts',(17.4122595410463,1.57578375247122,-6.64681501561899));
#12126=CARTESIAN_POINT('Ctrl Pts',(18.8002236181422,2.1943040052823,-4.51505601963387));
#12127=CARTESIAN_POINT('Ctrl Pts',(19.2902956110326,2.44248890127282,-3.32400070588094));
#12128=CARTESIAN_POINT('Ctrl Pts',(19.7901343922786,2.696799472177,-0.863253693613933));
#12129=CARTESIAN_POINT('Ctrl Pts',(19.8198403086391,2.71274440835119,0.36216566135821));
#12130=CARTESIAN_POINT('Ctrl Pts',(19.450604566805,2.52354005493898,2.7684762978899));
#12131=CARTESIAN_POINT('Ctrl Pts',(19.0587240926145,2.322406562892,3.91259636003955));
#12132=CARTESIAN_POINT('Ctrl Pts',(17.8594783884844,1.76766583827933,6.08297459859969));
#12133=CARTESIAN_POINT('Ctrl Pts',(17.0268766086191,1.40663102240569,7.07457363856991));
#12134=CARTESIAN_POINT('Ctrl Pts',(15.0677936986477,0.732379395365387,8.64898495762566));
#12135=CARTESIAN_POINT('Ctrl Pts',(13.9536542495791,0.421460567512847,9.24076616447532));
#12136=CARTESIAN_POINT('Ctrl Pts',(11.8519809404125,0.0796474466335174,
9.86534193353201));
#12137=CARTESIAN_POINT('Ctrl Pts',(10.9317093488347,0.000689942918333018,
10.0003289630384));
#12138=CARTESIAN_POINT('Ctrl Pts',(9.99999987317287,0.000194077067732486,
10.0000928969774));
#12139=CARTESIAN_POINT('Ctrl Pts',(10.,0.000187141247131616,9.99998766579631));
#12140=CARTESIAN_POINT('Ctrl Pts',(10.,10.7044979812508,9.29446313607499));
#12141=CARTESIAN_POINT('Ctrl Pts',(10.,20.2758418106305,4.44993914281691));
#12142=CARTESIAN_POINT('Origin',(24.,-17.3205080756888,4.50694379621148E-15));
#12143=CARTESIAN_POINT('',(13.7768139033962,1.77236952303898,5.955));
#12144=CARTESIAN_POINT('',(13.7768139033962,1.77236952303898,-5.955));
#12145=CARTESIAN_POINT('Origin',(13.7768139033962,-17.3205080756888,4.50694379621148E-15));
#12146=CARTESIAN_POINT('',(6.67681390339618,1.77236952303898,-5.955));
#12147=CARTESIAN_POINT('',(24.,1.77236952303898,-5.955));
#12148=CARTESIAN_POINT('',(6.67681390339617,1.77236952303898,5.955));
#12149=CARTESIAN_POINT('Origin',(6.67681390339618,-17.3205080756888,4.50694379621148E-15));
#12150=CARTESIAN_POINT('',(24.,1.77236952303898,5.955));
#12151=CARTESIAN_POINT('Origin',(0.,10.,0.));
#12152=CARTESIAN_POINT('',(13.7768139033962,10.,-5.955));
#12153=CARTESIAN_POINT('',(13.7768139033962,10.,5.955));
#12154=CARTESIAN_POINT('',(13.7768139033962,10.,5.955));
#12155=CARTESIAN_POINT('',(6.67681390339617,10.,5.955));
#12156=CARTESIAN_POINT('',(6.67681390339617,10.,5.955));
#12157=CARTESIAN_POINT('',(6.67681390339618,10.,-5.955));
#12158=CARTESIAN_POINT('',(6.67681390339617,10.,5.955));
#12159=CARTESIAN_POINT('',(6.67681390339618,10.,-5.955));
#12160=CARTESIAN_POINT('Origin',(6.67681390339617,10.,5.955));
#12161=CARTESIAN_POINT('',(6.67681390339617,10.,5.955));
#12162=CARTESIAN_POINT('',(13.7768139033962,10.,5.955));
#12163=CARTESIAN_POINT('Origin',(6.67681390339617,10.,5.955));
#12164=CARTESIAN_POINT('',(6.67681390339618,10.,-5.955));
#12165=CARTESIAN_POINT('Origin',(6.67681390339618,10.,-5.955));
#12166=CARTESIAN_POINT('',(13.7768139033962,10.,-5.955));
#12167=CARTESIAN_POINT('Origin',(13.7768139033962,10.,5.955));
#13164=UNCERTAINTY_MEASURE_WITH_UNIT(LENGTH_MEASURE(0.01),#13200,
'DISTANCE_ACCURACY_VALUE',
'Maximum model space distance between geometric entities at asserted c
onnectivities');
#13173=UNCERTAINTY_MEASURE_WITH_UNIT(LENGTH_MEASURE(0.01),#13200,
'DISTANCE_ACCURACY_VALUE',
'Maximum model space distance between geometric entities at asserted c
onnectivities');
#13190=(
GEOMETRIC_REPRESENTATION_CONTEXT(3)
GLOBAL_UNCERTAINTY_ASSIGNED_CONTEXT((#13164))
GLOBAL_UNIT_ASSIGNED_CONTEXT((#13200,#13202,#13203))
REPRESENTATION_CONTEXT('','3D')
);
#13199=(
GEOMETRIC_REPRESENTATION_CONTEXT(3)
GLOBAL_UNCERTAINTY_ASSIGNED_CONTEXT((#13173))
GLOBAL_UNIT_ASSIGNED_CONTEXT((#13200,#13202,#13203))
REPRESENTATION_CONTEXT('','3D')
);
#13200=(
LENGTH_UNIT()
NAMED_UNIT(*)
SI_UNIT(.MILLI.,.METRE.)
);
#13202=(
NAMED_UNIT(*)
PLANE_ANGLE_UNIT()
SI_UNIT($,.RADIAN.)
);
#13203=(
NAMED_UNIT(*)
SI_UNIT($,.STERADIAN.)
SOLID_ANGLE_UNIT()
);
#13220=SHAPE_DEFINITION_REPRESENTATION(#13252,#13294);
#13252=PRODUCT_DEFINITION_SHAPE('',$,#13320);
#13294=SHAPE_REPRESENTATION('',(#7595),#13190);
#13303=PRODUCT_DEFINITION_CONTEXT('part definition',#13380,'design');
#13320=PRODUCT_DEFINITION('Finger Tip','Finger Tip',#13345,#13303);
#13345=PRODUCT_DEFINITION_FORMATION('',$,#13398);
#13380=APPLICATION_CONTEXT(
'Core Data for Automotive Mechanical Design Process');
#13381=PRODUCT_CONTEXT('part definition',#13380,'mechanical');
#13398=PRODUCT('Finger Tip','Finger Tip',$,(#13381));
#13409=PRESENTATION_STYLE_ASSIGNMENT((#13414));
#13414=SURFACE_STYLE_USAGE(.BOTH.,#13419);
#13419=SURFACE_SIDE_STYLE('',(#13424));
#13424=SURFACE_STYLE_FILL_AREA(#13429);
#13429=FILL_AREA_STYLE('Opaque(61,176,222)',(#13434));
#13434=FILL_AREA_STYLE_COLOUR('Opaque(61,176,222)',#13439);
#13439=COLOUR_RGB('Opaque(61,176,222)',0.23921568627451,0.690196078431373,
0.870588235294118);
ENDSEC;
END-ISO-10303-21;
